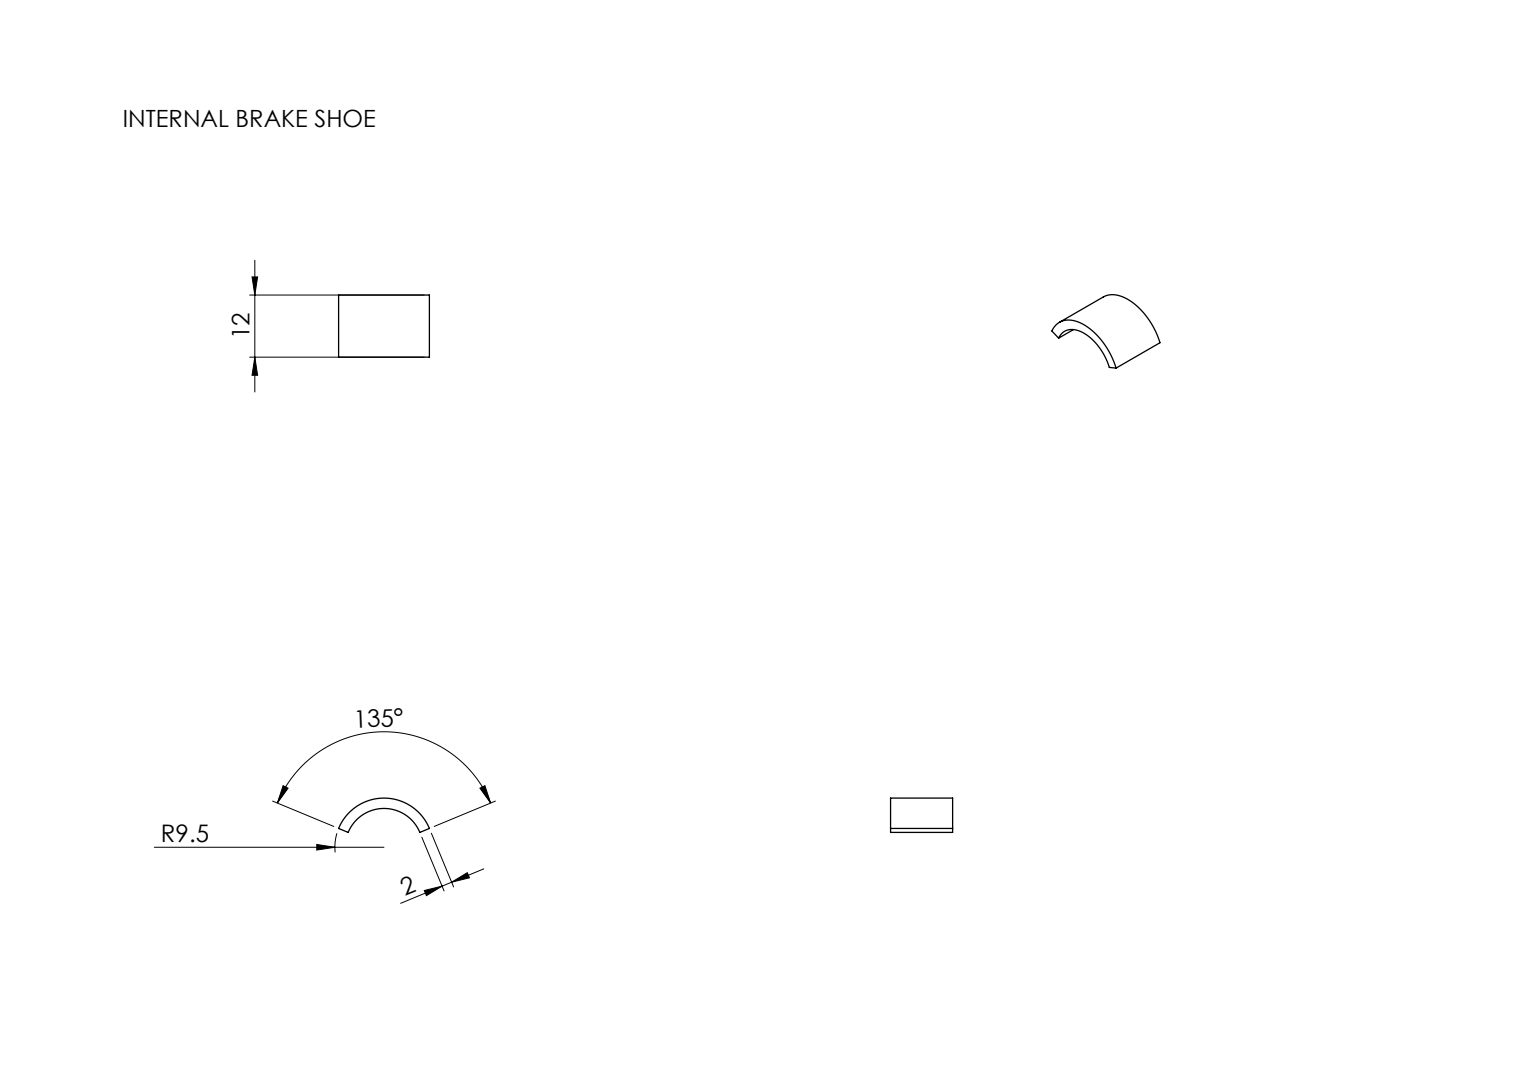
ISO-10303-21;
HEADER;
FILE_DESCRIPTION (('STEP AP214'),
    '1' );
FILE_NAME ('Internal Brake Shoe.step',
    '2026-10-08T05:56:58',
    ( '' ),
    ( '' ),
    'SwSTEP 2.0',
    'SolidWorks 2026',
    '' );
FILE_SCHEMA (( 'AUTOMOTIVE_DESIGN' ));
ENDSEC;

DATA;
#60=FILL_AREA_STYLE ('',( #15279 ) ) ;
#126=VERTEX_POINT ( 'NONE', #442 ) ;
#199=SURFACE_SIDE_STYLE ('',( #8289 ) ) ;
#301=FACE_OUTER_BOUND ( 'NONE', #19198, .T. ) ;
#391=( NAMED_UNIT ( * ) PLANE_ANGLE_UNIT ( ) SI_UNIT ( $, .RADIAN. ) );
#411=VERTEX_POINT ( 'NONE', #14043 ) ;
#442=CARTESIAN_POINT ( 'NONE',  ( -6.929096493834647319, 2.870125742738179664, 12.00000000000000000 ) ) ;
#578=ORIENTED_EDGE ( 'NONE', *, *, #10615, .F. ) ;
#594=CARTESIAN_POINT ( 'NONE',  ( 0.000000000000000000, 0.000000000000000000, 12.00000000000000000 ) ) ;
#695=PRESENTATION_STYLE_ASSIGNMENT (( #7886 ) ) ;
#788=DIRECTION ( 'NONE',  ( 1.000000000000000000, 0.000000000000000000, -0.000000000000000000 ) ) ;
#793=DIRECTION ( 'NONE',  ( -1.000000000000000000, 0.000000000000000000, 0.000000000000000000 ) ) ;
#827=CARTESIAN_POINT ( 'NONE',  ( 8.776855558857221240, 3.635492607468361559, 0.000000000000000000 ) ) ;
#886=DIRECTION ( 'NONE',  ( -0.000000000000000000, -0.000000000000000000, -1.000000000000000000 ) ) ;
#1241=ADVANCED_FACE ( 'NONE', ( #2565 ), #8492, .T. ) ;
#1407=CARTESIAN_POINT ( 'NONE',  ( 0.000000000000000000, 0.000000000000000000, 0.000000000000000000 ) ) ;
#1533=VERTEX_POINT ( 'NONE', #5432 ) ;
#1574=CARTESIAN_POINT ( 'NONE',  ( -6.929096493834647319, 2.870125742738179664, 12.00000000000000000 ) ) ;
#1727=DIRECTION ( 'NONE',  ( -1.000000000000000000, 0.000000000000000000, 0.000000000000000000 ) ) ;
#1753=SHAPE_DEFINITION_REPRESENTATION ( #11783, #7967 ) ;
#1762=CIRCLE ( 'NONE', #19009, 9.500000000000000000 ) ;
#1784=LINE ( 'NONE', #18588, #6227 ) ;
#1891=CARTESIAN_POINT ( 'NONE',  ( 6.929096493834647319, 2.870125742738179664, 0.000000000000000000 ) ) ;
#1896=CARTESIAN_POINT ( 'NONE',  ( 8.776855558857221240, 3.635492607468361559, 12.00000000000000000 ) ) ;
#1915=FACE_OUTER_BOUND ( 'NONE', #6557, .T. ) ;
#2059=EDGE_CURVE ( 'NONE', #1533, #12097, #1762, .T. ) ;
#2102=CARTESIAN_POINT ( 'NONE',  ( 0.000000000000000000, 0.000000000000000000, 0.000000000000000000 ) ) ;
#2185=FILL_AREA_STYLE ('',( #3686 ) ) ;
#2320=STYLED_ITEM ( 'NONE', ( #4664 ), #9128 ) ;
#2565=FACE_OUTER_BOUND ( 'NONE', #14746, .T. ) ;
#2573=UNCERTAINTY_MEASURE_WITH_UNIT (LENGTH_MEASURE( 1.000000000000000082E-05 ), #5287, 'distance_accuracy_value', 'NONE');
#2873=ADVANCED_FACE ( 'NONE', ( #3246 ), #6333, .T. ) ;
#2978=DIRECTION ( 'NONE',  ( -0.000000000000000000, -0.000000000000000000, -1.000000000000000000 ) ) ;
#3221=CYLINDRICAL_SURFACE ( 'NONE', #4163, 7.500000000000000000 ) ;
#3246=FACE_OUTER_BOUND ( 'NONE', #3907, .T. ) ;
#3453=VERTEX_POINT ( 'NONE', #9388 ) ;
#3460=VECTOR ( 'NONE', #19558, 1000.000000000000000 ) ;
#3568=DIRECTION ( 'NONE',  ( 1.000000000000000000, 0.000000000000000000, 0.000000000000000000 ) ) ;
#3671=EDGE_CURVE ( 'NONE', #411, #1533, #5321, .T. ) ;
#3686=FILL_AREA_STYLE_COLOUR ( '', #7128 ) ;
#3850=ORIENTED_EDGE ( 'NONE', *, *, #5946, .T. ) ;
#3873=CARTESIAN_POINT ( 'NONE',  ( 0.000000000000000000, 0.000000000000000000, 0.000000000000000000 ) ) ;
#3907=EDGE_LOOP ( 'NONE', ( #15439, #5683, #14430, #10674 ) ) ;
#4163=AXIS2_PLACEMENT_3D ( 'NONE', #18528, #8011, #1727 ) ;
#4346=VECTOR ( 'NONE', #14837, 999.9999999999998863 ) ;
#4632=CARTESIAN_POINT ( 'NONE',  ( 6.929096493834647319, 2.870125742738179664, 12.00000000000000000 ) ) ;
#4664=PRESENTATION_STYLE_ASSIGNMENT (( #18371 ) ) ;
#4770=LINE ( 'NONE', #1574, #18756 ) ;
#4807=AXIS2_PLACEMENT_3D ( 'NONE', #1896, #13808, #10907 ) ;
#4991=( NAMED_UNIT ( * ) SI_UNIT ( $, .STERADIAN. ) SOLID_ANGLE_UNIT ( ) );
#5016=VECTOR ( 'NONE', #5602, 1000.000000000000114 ) ;
#5097=DIRECTION ( 'NONE',  ( 1.000000000000000000, 0.000000000000000000, 0.000000000000000000 ) ) ;
#5287=( LENGTH_UNIT ( ) NAMED_UNIT ( * ) SI_UNIT ( .MILLI., .METRE. ) );
#5321=LINE ( 'NONE', #17532, #5016 ) ;
#5389=DIRECTION ( 'NONE',  ( 0.000000000000000000, 0.000000000000000000, 1.000000000000000000 ) ) ;
#5432=CARTESIAN_POINT ( 'NONE',  ( -8.776855558857221240, 3.635492607468361115, 0.000000000000000000 ) ) ;
#5481=PLANE ( 'NONE',  #6077 ) ;
#5541=ORIENTED_EDGE ( 'NONE', *, *, #16918, .T. ) ;
#5556=CARTESIAN_POINT ( 'NONE',  ( -6.929096493834647319, 2.870125742738179664, 12.00000000000000000 ) ) ;
#5602=DIRECTION ( 'NONE',  ( -0.9238795325112865164, 0.3826834323650905034, 0.000000000000000000 ) ) ;
#5683=ORIENTED_EDGE ( 'NONE', *, *, #13076, .F. ) ;
#5887=ADVANCED_BREP_SHAPE_REPRESENTATION ( '', ( #9128, #16724 ), #6818 ) ;
#5946=EDGE_CURVE ( 'NONE', #411, #11096, #8513, .T. ) ;
#6077=AXIS2_PLACEMENT_3D ( 'NONE', #19095, #5389, #7067 ) ;
#6154=SURFACE_STYLE_FILL_AREA ( #60 ) ;
#6227=VECTOR ( 'NONE', #11089, 1000.000000000000000 ) ;
#6230=DIRECTION ( 'NONE',  ( 1.000000000000000000, 0.000000000000000000, 0.000000000000000000 ) ) ;
#6293=ORIENTED_EDGE ( 'NONE', *, *, #2059, .F. ) ;
#6333=PLANE ( 'NONE',  #14479 ) ;
#6440=CIRCLE ( 'NONE', #7396, 7.500000000000000000 ) ;
#6508=AXIS2_PLACEMENT_3D ( 'NONE', #594, #886, #793 ) ;
#6538=( NAMED_UNIT ( * ) SI_UNIT ( $, .STERADIAN. ) SOLID_ANGLE_UNIT ( ) );
#6557=EDGE_LOOP ( 'NONE', ( #3850, #9763, #13981, #16885 ) ) ;
#6663=DIRECTION ( 'NONE',  ( 0.000000000000000000, 0.000000000000000000, 1.000000000000000000 ) ) ;
#6757=DIRECTION ( 'NONE',  ( -0.000000000000000000, -0.000000000000000000, -1.000000000000000000 ) ) ;
#6818=( GEOMETRIC_REPRESENTATION_CONTEXT ( 3 ) GLOBAL_UNCERTAINTY_ASSIGNED_CONTEXT ( ( #8591 ) ) GLOBAL_UNIT_ASSIGNED_CONTEXT ( ( #14093, #391, #4991 ) ) REPRESENTATION_CONTEXT ( 'NONE', 'WORKASPACE' ) );
#7067=DIRECTION ( 'NONE',  ( 1.000000000000000000, 0.000000000000000000, -0.000000000000000000 ) ) ;
#7128=COLOUR_RGB ( '', 0.08235294, 0.09019608, 0.10196078) ;
#7322=ORIENTED_EDGE ( 'NONE', *, *, #18492, .T. ) ;
#7338=LINE ( 'NONE', #5556, #3460 ) ;
#7396=AXIS2_PLACEMENT_3D ( 'NONE', #19074, #6757, #3568 ) ;
#7409=VECTOR ( 'NONE', #19256, 1000.000000000000000 ) ;
#7488=DIRECTION ( 'NONE',  ( -0.000000000000000000, -0.000000000000000000, -1.000000000000000000 ) ) ;
#7515=ORIENTED_EDGE ( 'NONE', *, *, #5946, .F. ) ;
#7711=EDGE_CURVE ( 'NONE', #126, #3453, #6440, .T. ) ;
#7843=DIRECTION ( 'NONE',  ( 0.9238795325112865164, -0.3826834323650905034, 0.000000000000000000 ) ) ;
#7886=SURFACE_STYLE_USAGE ( .BOTH. , #199 ) ;
#7967=SHAPE_REPRESENTATION ( 'Internal Brake Shoe', ( #16724 ), #6818 ) ;
#8011=DIRECTION ( 'NONE',  ( -0.000000000000000000, -0.000000000000000000, -1.000000000000000000 ) ) ;
#8289=SURFACE_STYLE_FILL_AREA ( #2185 ) ;
#8304=DIRECTION ( 'NONE',  ( -0.000000000000000000, -0.000000000000000000, -1.000000000000000000 ) ) ;
#8428=MECHANICAL_DESIGN_GEOMETRIC_PRESENTATION_REPRESENTATION('',(#9723),#12267);
#8467=ORIENTED_EDGE ( 'NONE', *, *, #7711, .T. ) ;
#8492=CYLINDRICAL_SURFACE ( 'NONE', #6508, 9.500000000000000000 ) ;
#8513=CIRCLE ( 'NONE', #16187, 7.500000000000000000 ) ;
#8591=UNCERTAINTY_MEASURE_WITH_UNIT (LENGTH_MEASURE( 1.000000000000000082E-05 ), #14093, 'distance_accuracy_value', 'NONE');
#8868=ORIENTED_EDGE ( 'NONE', *, *, #13771, .T. ) ;
#9069=APPLICATION_CONTEXT ( 'automotive_design' ) ;
#9128=MANIFOLD_SOLID_BREP ( 'Extrude-Thin1', #11952 ) ;
#9361=DIRECTION ( 'NONE',  ( -0.3826834323650905034, -0.9238795325112865164, 0.000000000000000000 ) ) ;
#9388=CARTESIAN_POINT ( 'NONE',  ( 6.929096493834647319, 2.870125742738179664, 12.00000000000000000 ) ) ;
#9409=DIRECTION ( 'NONE',  ( -1.000000000000000000, 0.000000000000000000, 0.000000000000000000 ) ) ;
#9651=EDGE_CURVE ( 'NONE', #14843, #1533, #1784, .T. ) ;
#9723=STYLED_ITEM ( 'NONE', ( #695 ), #5887 ) ;
#9763=ORIENTED_EDGE ( 'NONE', *, *, #13771, .F. ) ;
#9800=PLANE ( 'NONE',  #16463 ) ;
#9833=DIRECTION ( 'NONE',  ( 0.000000000000000000, 0.000000000000000000, 1.000000000000000000 ) ) ;
#9834=ADVANCED_FACE ( 'NONE', ( #14289 ), #9800, .F. ) ;
#9940=CIRCLE ( 'NONE', #17272, 9.500000000000000000 ) ;
#10200=PRODUCT_DEFINITION_FORMATION_WITH_SPECIFIED_SOURCE ( 'ANY', '', #17690, .NOT_KNOWN. ) ;
#10328=CARTESIAN_POINT ( 'NONE',  ( 8.776855558857221240, 3.635492607468361559, 12.00000000000000000 ) ) ;
#10532=LINE ( 'NONE', #18043, #4346 ) ;
#10585=DIRECTION ( 'NONE',  ( -0.9238795325112865164, 0.3826834323650905034, 0.000000000000000000 ) ) ;
#10615=EDGE_CURVE ( 'NONE', #16727, #3453, #10532, .T. ) ;
#10674=ORIENTED_EDGE ( 'NONE', *, *, #9651, .T. ) ;
#10899=PRODUCT_DEFINITION ( 'UNKNOWN', '', #10200, #13587 ) ;
#10907=DIRECTION ( 'NONE',  ( 0.9238795325112864054, 0.3826834323650906700, 0.000000000000000000 ) ) ;
#10922=LINE ( 'NONE', #11119, #12837 ) ;
#10951=COLOUR_RGB ( '', 0.08235294, 0.09019608, 0.10196078) ;
#11089=DIRECTION ( 'NONE',  ( -0.000000000000000000, -0.000000000000000000, -1.000000000000000000 ) ) ;
#11096=VERTEX_POINT ( 'NONE', #1891 ) ;
#11119=CARTESIAN_POINT ( 'NONE',  ( 8.776855558857221240, 3.635492607468361559, 0.000000000000000000 ) ) ;
#11310=DIRECTION ( 'NONE',  ( -0.000000000000000000, -0.000000000000000000, -1.000000000000000000 ) ) ;
#11581=EDGE_CURVE ( 'NONE', #126, #14843, #4770, .T. ) ;
#11783=PRODUCT_DEFINITION_SHAPE ( 'NONE', 'NONE',  #10899 ) ;
#11863=EDGE_LOOP ( 'NONE', ( #7515, #17958, #14662, #7322 ) ) ;
#11902=( GEOMETRIC_REPRESENTATION_CONTEXT ( 3 ) GLOBAL_UNCERTAINTY_ASSIGNED_CONTEXT ( ( #19188 ) ) GLOBAL_UNIT_ASSIGNED_CONTEXT ( ( #14367, #12671, #6538 ) ) REPRESENTATION_CONTEXT ( 'NONE', 'WORKASPACE' ) );
#11952=CLOSED_SHELL ( 'NONE', ( #15535, #16769, #1241, #2873, #16855, #9834 ) ) ;
#12097=VERTEX_POINT ( 'NONE', #827 ) ;
#12132=APPLICATION_CONTEXT ( 'automotive_design' ) ;
#12267=( GEOMETRIC_REPRESENTATION_CONTEXT ( 3 ) GLOBAL_UNCERTAINTY_ASSIGNED_CONTEXT ( ( #2573 ) ) GLOBAL_UNIT_ASSIGNED_CONTEXT ( ( #5287, #12898, #17888 ) ) REPRESENTATION_CONTEXT ( 'NONE', 'WORKASPACE' ) );
#12272=SURFACE_SIDE_STYLE ('',( #6154 ) ) ;
#12671=( NAMED_UNIT ( * ) PLANE_ANGLE_UNIT ( ) SI_UNIT ( $, .RADIAN. ) );
#12837=VECTOR ( 'NONE', #17027, 999.9999999999998863 ) ;
#12871=CARTESIAN_POINT ( 'NONE',  ( -8.776855558857221240, 3.635492607468361115, 12.00000000000000000 ) ) ;
#12898=( NAMED_UNIT ( * ) PLANE_ANGLE_UNIT ( ) SI_UNIT ( $, .RADIAN. ) );
#13076=EDGE_CURVE ( 'NONE', #126, #411, #7338, .T. ) ;
#13165=CARTESIAN_POINT ( 'NONE',  ( 8.776855558857221240, 3.635492607468361559, 12.00000000000000000 ) ) ;
#13239=ORIENTED_EDGE ( 'NONE', *, *, #16918, .F. ) ;
#13275=ORIENTED_EDGE ( 'NONE', *, *, #10615, .T. ) ;
#13587=PRODUCT_DEFINITION_CONTEXT ( 'detailed design', #9069, 'design' ) ;
#13771=EDGE_CURVE ( 'NONE', #3453, #11096, #18342, .T. ) ;
#13808=DIRECTION ( 'NONE',  ( 0.3826834323650906700, -0.9238795325112864054, 0.000000000000000000 ) ) ;
#13981=ORIENTED_EDGE ( 'NONE', *, *, #7711, .F. ) ;
#14043=CARTESIAN_POINT ( 'NONE',  ( -6.929096493834647319, 2.870125742738179664, 0.000000000000000000 ) ) ;
#14093=( LENGTH_UNIT ( ) NAMED_UNIT ( * ) SI_UNIT ( .MILLI., .METRE. ) );
#14289=FACE_OUTER_BOUND ( 'NONE', #11863, .T. ) ;
#14367=( LENGTH_UNIT ( ) NAMED_UNIT ( * ) SI_UNIT ( .MILLI., .METRE. ) );
#14430=ORIENTED_EDGE ( 'NONE', *, *, #11581, .T. ) ;
#14479=AXIS2_PLACEMENT_3D ( 'NONE', #18455, #9361, #7843 ) ;
#14662=ORIENTED_EDGE ( 'NONE', *, *, #2059, .T. ) ;
#14746=EDGE_LOOP ( 'NONE', ( #6293, #16244, #5541, #15046 ) ) ;
#14837=DIRECTION ( 'NONE',  ( -0.9238795325112865164, -0.3826834323650906700, 0.000000000000000000 ) ) ;
#14843=VERTEX_POINT ( 'NONE', #12871 ) ;
#15046=ORIENTED_EDGE ( 'NONE', *, *, #19542, .T. ) ;
#15279=FILL_AREA_STYLE_COLOUR ( '', #10951 ) ;
#15382=ORIENTED_EDGE ( 'NONE', *, *, #18492, .F. ) ;
#15439=ORIENTED_EDGE ( 'NONE', *, *, #3671, .F. ) ;
#15535=ADVANCED_FACE ( 'NONE', ( #1915 ), #3221, .F. ) ;
#15558=PRODUCT_CONTEXT ( 'NONE', #12132, 'mechanical' ) ;
#15873=LINE ( 'NONE', #13165, #7409 ) ;
#16001=CARTESIAN_POINT ( 'NONE',  ( 0.000000000000000000, 0.000000000000000000, 12.00000000000000000 ) ) ;
#16187=AXIS2_PLACEMENT_3D ( 'NONE', #2102, #8304, #5097 ) ;
#16244=ORIENTED_EDGE ( 'NONE', *, *, #9651, .F. ) ;
#16251=EDGE_LOOP ( 'NONE', ( #8467, #578, #13239, #19396 ) ) ;
#16397=DIRECTION ( 'NONE',  ( -1.000000000000000000, 0.000000000000000000, 0.000000000000000000 ) ) ;
#16463=AXIS2_PLACEMENT_3D ( 'NONE', #3873, #6663, #788 ) ;
#16724=AXIS2_PLACEMENT_3D ( 'NONE', #17428, #9833, #6230 ) ;
#16727=VERTEX_POINT ( 'NONE', #10328 ) ;
#16769=ADVANCED_FACE ( 'NONE', ( #301 ), #16919, .T. ) ;
#16855=ADVANCED_FACE ( 'NONE', ( #19189 ), #5481, .T. ) ;
#16885=ORIENTED_EDGE ( 'NONE', *, *, #13076, .T. ) ;
#16918=EDGE_CURVE ( 'NONE', #14843, #16727, #9940, .T. ) ;
#16919=PLANE ( 'NONE',  #4807 ) ;
#17027=DIRECTION ( 'NONE',  ( -0.9238795325112865164, -0.3826834323650906700, 0.000000000000000000 ) ) ;
#17272=AXIS2_PLACEMENT_3D ( 'NONE', #16001, #2978, #16397 ) ;
#17428=CARTESIAN_POINT ( 'NONE',  ( 0.000000000000000000, 0.000000000000000000, 0.000000000000000000 ) ) ;
#17532=CARTESIAN_POINT ( 'NONE',  ( -6.929096493834647319, 2.870125742738179664, 0.000000000000000000 ) ) ;
#17690=PRODUCT ( 'Internal Brake Shoe', 'Internal Brake Shoe', '', ( #15558 ) ) ;
#17736=ORIENTED_EDGE ( 'NONE', *, *, #19542, .F. ) ;
#17888=( NAMED_UNIT ( * ) SI_UNIT ( $, .STERADIAN. ) SOLID_ANGLE_UNIT ( ) );
#17958=ORIENTED_EDGE ( 'NONE', *, *, #3671, .T. ) ;
#17981=MECHANICAL_DESIGN_GEOMETRIC_PRESENTATION_REPRESENTATION('',(#2320),#11902);
#18043=CARTESIAN_POINT ( 'NONE',  ( 8.776855558857221240, 3.635492607468361559, 12.00000000000000000 ) ) ;
#18342=LINE ( 'NONE', #4632, #18511 ) ;
#18371=SURFACE_STYLE_USAGE ( .BOTH. , #12272 ) ;
#18455=CARTESIAN_POINT ( 'NONE',  ( -6.929096493834647319, 2.870125742738179664, 12.00000000000000000 ) ) ;
#18492=EDGE_CURVE ( 'NONE', #12097, #11096, #10922, .T. ) ;
#18511=VECTOR ( 'NONE', #11310, 1000.000000000000000 ) ;
#18528=CARTESIAN_POINT ( 'NONE',  ( 0.000000000000000000, 0.000000000000000000, 12.00000000000000000 ) ) ;
#18588=CARTESIAN_POINT ( 'NONE',  ( -8.776855558857221240, 3.635492607468361115, 12.00000000000000000 ) ) ;
#18756=VECTOR ( 'NONE', #10585, 1000.000000000000114 ) ;
#18995=SHAPE_REPRESENTATION_RELATIONSHIP ( 'NONE' , 'NONE' ,  #7967, #5887 ) ;
#19009=AXIS2_PLACEMENT_3D ( 'NONE', #1407, #7488, #9409 ) ;
#19074=CARTESIAN_POINT ( 'NONE',  ( 0.000000000000000000, 0.000000000000000000, 12.00000000000000000 ) ) ;
#19095=CARTESIAN_POINT ( 'NONE',  ( 0.000000000000000000, 0.000000000000000000, 12.00000000000000000 ) ) ;
#19188=UNCERTAINTY_MEASURE_WITH_UNIT (LENGTH_MEASURE( 1.000000000000000082E-05 ), #14367, 'distance_accuracy_value', 'NONE');
#19189=FACE_OUTER_BOUND ( 'NONE', #16251, .T. ) ;
#19198=EDGE_LOOP ( 'NONE', ( #15382, #17736, #13275, #8868 ) ) ;
#19256=DIRECTION ( 'NONE',  ( -0.000000000000000000, -0.000000000000000000, -1.000000000000000000 ) ) ;
#19396=ORIENTED_EDGE ( 'NONE', *, *, #11581, .F. ) ;
#19542=EDGE_CURVE ( 'NONE', #16727, #12097, #15873, .T. ) ;
#19558=DIRECTION ( 'NONE',  ( -0.000000000000000000, -0.000000000000000000, -1.000000000000000000 ) ) ;
ENDSEC;
END-ISO-10303-21;
